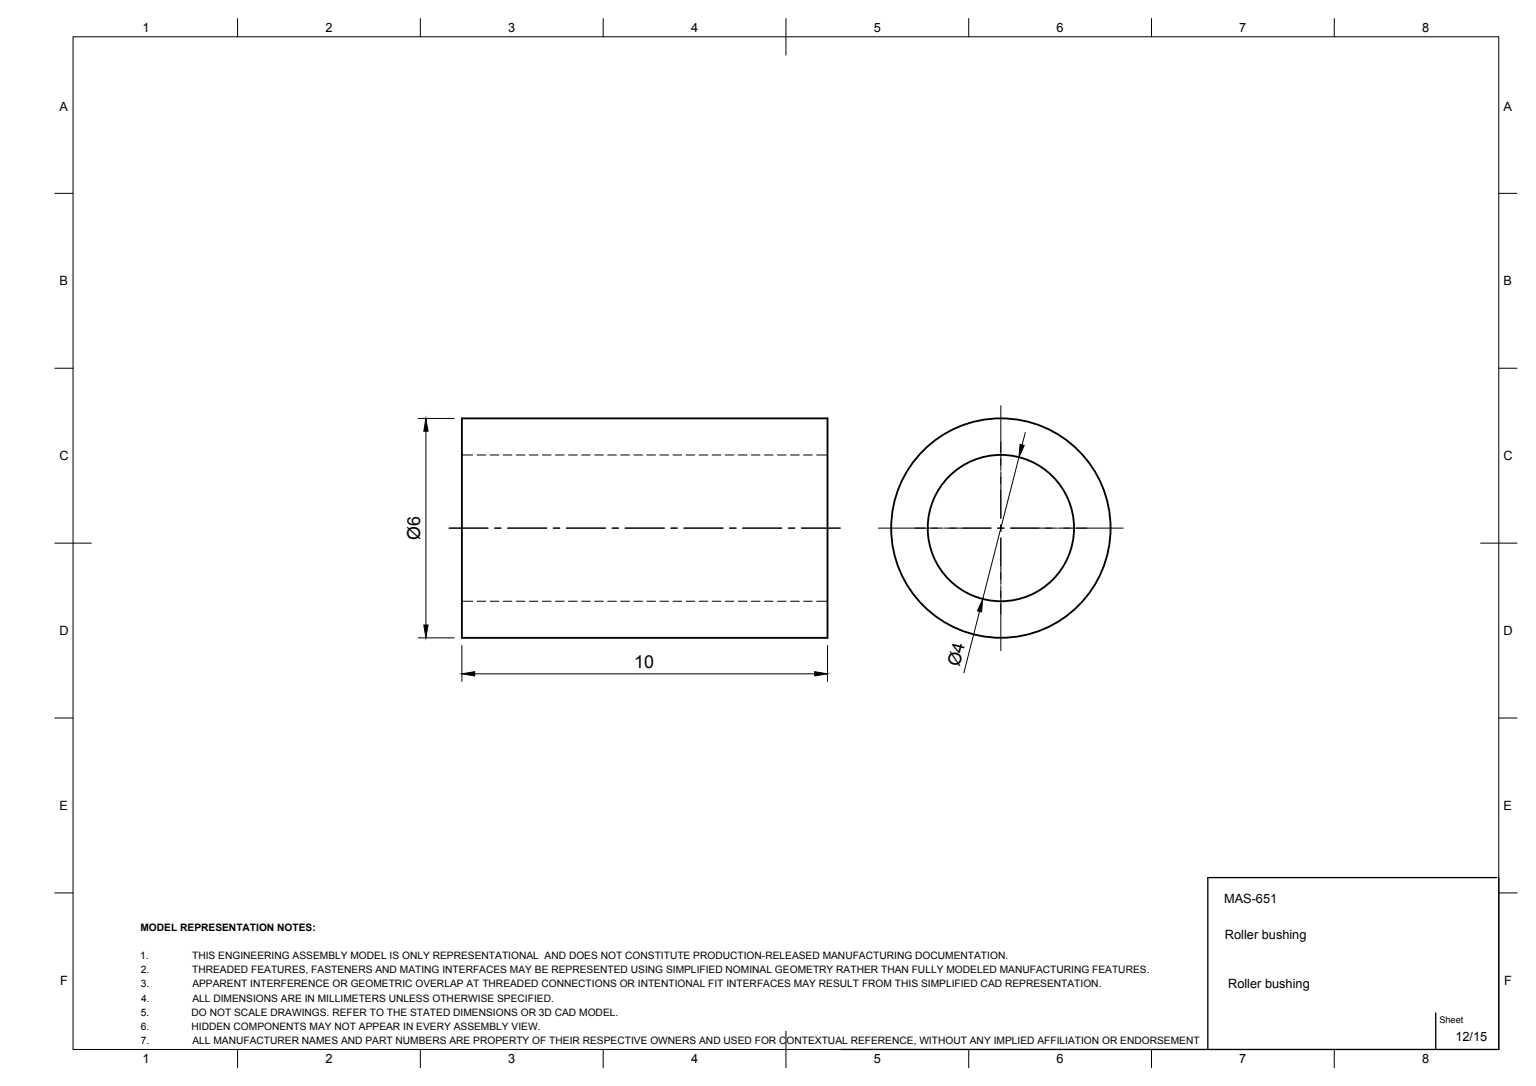
ISO-10303-21;
HEADER;
/* Generated by software containing ST-Developer
 * from STEP Tools, Inc. (www.steptools.com) 
 */

FILE_DESCRIPTION(
/* description */ ('Independent direct-acting normally-closed roller-plunger limit-switch
 CAD. Removable cover, insulated terminal supports, captured bus/conta
ct bridge, native Coil return spring, integral lower travel stop, reus
able instanced hardware and free roller. Manual geometric contact open
ing4mm; no snap-action/contact-force, electrical/current/voltage, envi
ronmental seal, safety-switch, wear, load or life certification. Exter
nal wiring and anchors omitted; fits and application engineering requi
red.'),
/* implementation_level */ '2;1');

FILE_NAME(
/* name */ 'Roller bushing.step',
/* time_stamp */ '2026-11-08T07:32:43-08:00',
/* author */ (''),
/* organization */ (''),
/* preprocessor_version */ 'ST-DEVELOPER v20.2',
/* originating_system */ 'Autodesk Translation Framework v15.17.0.0',
/* authorisation */ '');

FILE_SCHEMA (('AUTOMOTIVE_DESIGN { 1 0 10303 214 3 1 1 }'));
ENDSEC;

DATA;
#10=MECHANICAL_DESIGN_GEOMETRIC_PRESENTATION_REPRESENTATION('',(#185),#36482);
#151=SHAPE_REPRESENTATION_RELATIONSHIP('SRR','None',#36564,#168);
#168=ADVANCED_BREP_SHAPE_REPRESENTATION('',(#202),#36474);
#185=STYLED_ITEM('',(#36657),#202);
#202=MANIFOLD_SOLID_BREP('Body1',#9776);
#289=FACE_BOUND('',#1410,.T.);
#290=FACE_BOUND('',#1412,.T.);
#394=PLANE('',#10460);
#395=PLANE('',#10461);
#815=FACE_OUTER_BOUND('',#1407,.T.);
#816=FACE_OUTER_BOUND('',#1408,.T.);
#817=FACE_OUTER_BOUND('',#1409,.T.);
#818=FACE_OUTER_BOUND('',#1411,.T.);
#1407=EDGE_LOOP('',(#8038,#8039,#8040,#8041));
#1408=EDGE_LOOP('',(#8042,#8043,#8044,#8045));
#1409=EDGE_LOOP('',(#8046));
#1410=EDGE_LOOP('',(#8047));
#1411=EDGE_LOOP('',(#8048));
#1412=EDGE_LOOP('',(#8049));
#1695=CIRCLE('',#10455,0.2);
#1696=CIRCLE('',#10456,0.2);
#1697=CIRCLE('',#10458,0.3);
#1698=CIRCLE('',#10459,0.3);
#2855=LINE('',#29247,#3429);
#2856=LINE('',#29253,#3430);
#3429=VECTOR('',#12068,0.2);
#3430=VECTOR('',#12075,0.3);
#4275=VERTEX_POINT('',#29244);
#4276=VERTEX_POINT('',#29246);
#4277=VERTEX_POINT('',#29250);
#4278=VERTEX_POINT('',#29252);
#5575=EDGE_CURVE('',#4275,#4275,#1695,.T.);
#5576=EDGE_CURVE('',#4275,#4276,#2855,.T.);
#5577=EDGE_CURVE('',#4276,#4276,#1696,.T.);
#5578=EDGE_CURVE('',#4277,#4277,#1697,.T.);
#5579=EDGE_CURVE('',#4277,#4278,#2856,.T.);
#5580=EDGE_CURVE('',#4278,#4278,#1698,.T.);
#8038=ORIENTED_EDGE('',*,*,#5575,.F.);
#8039=ORIENTED_EDGE('',*,*,#5576,.T.);
#8040=ORIENTED_EDGE('',*,*,#5577,.T.);
#8041=ORIENTED_EDGE('',*,*,#5576,.F.);
#8042=ORIENTED_EDGE('',*,*,#5578,.F.);
#8043=ORIENTED_EDGE('',*,*,#5579,.T.);
#8044=ORIENTED_EDGE('',*,*,#5580,.T.);
#8045=ORIENTED_EDGE('',*,*,#5579,.F.);
#8046=ORIENTED_EDGE('',*,*,#5578,.T.);
#8047=ORIENTED_EDGE('',*,*,#5575,.T.);
#8048=ORIENTED_EDGE('',*,*,#5580,.F.);
#8049=ORIENTED_EDGE('',*,*,#5577,.F.);
#9122=CYLINDRICAL_SURFACE('',#10454,0.2);
#9123=CYLINDRICAL_SURFACE('',#10457,0.3);
#9605=ADVANCED_FACE('',(#815),#9122,.F.);
#9606=ADVANCED_FACE('',(#816),#9123,.T.);
#9607=ADVANCED_FACE('',(#817,#289),#394,.T.);
#9608=ADVANCED_FACE('',(#818,#290),#395,.F.);
#9776=CLOSED_SHELL('',(#9605,#9606,#9607,#9608));
#10453=AXIS2_PLACEMENT_3D('',#29242,#12062,#12063);
#10454=AXIS2_PLACEMENT_3D('',#29243,#12064,#12065);
#10455=AXIS2_PLACEMENT_3D('',#29245,#12066,#12067);
#10456=AXIS2_PLACEMENT_3D('',#29248,#12069,#12070);
#10457=AXIS2_PLACEMENT_3D('',#29249,#12071,#12072);
#10458=AXIS2_PLACEMENT_3D('',#29251,#12073,#12074);
#10459=AXIS2_PLACEMENT_3D('',#29254,#12076,#12077);
#10460=AXIS2_PLACEMENT_3D('',#29255,#12078,#12079);
#10461=AXIS2_PLACEMENT_3D('',#29256,#12080,#12081);
#12062=DIRECTION('axis',(0.,0.,1.));
#12063=DIRECTION('refdir',(1.,0.,0.));
#12064=DIRECTION('center_axis',(0.,0.,1.));
#12065=DIRECTION('ref_axis',(1.,0.,0.));
#12066=DIRECTION('center_axis',(0.,0.,-1.));
#12067=DIRECTION('ref_axis',(1.,0.,0.));
#12068=DIRECTION('',(0.,0.,-1.));
#12069=DIRECTION('center_axis',(0.,0.,-1.));
#12070=DIRECTION('ref_axis',(1.,0.,0.));
#12071=DIRECTION('center_axis',(0.,0.,1.));
#12072=DIRECTION('ref_axis',(1.,0.,0.));
#12073=DIRECTION('center_axis',(0.,0.,1.));
#12074=DIRECTION('ref_axis',(1.,0.,0.));
#12075=DIRECTION('',(0.,0.,-1.));
#12076=DIRECTION('center_axis',(0.,0.,1.));
#12077=DIRECTION('ref_axis',(1.,0.,0.));
#12078=DIRECTION('center_axis',(0.,0.,1.));
#12079=DIRECTION('ref_axis',(1.,0.,0.));
#12080=DIRECTION('center_axis',(0.,0.,1.));
#12081=DIRECTION('ref_axis',(1.,0.,0.));
#29242=CARTESIAN_POINT('',(0.,0.,0.));
#29243=CARTESIAN_POINT('Origin',(0.,0.,0.));
#29244=CARTESIAN_POINT('',(-0.2,-2.44929359829471E-17,1.));
#29245=CARTESIAN_POINT('Origin',(0.,0.,1.));
#29246=CARTESIAN_POINT('',(-0.2,-2.44929359829471E-17,0.));
#29247=CARTESIAN_POINT('',(-0.2,-2.44929359829471E-17,0.));
#29248=CARTESIAN_POINT('Origin',(0.,0.,0.));
#29249=CARTESIAN_POINT('Origin',(0.,0.,0.));
#29250=CARTESIAN_POINT('',(-0.3,-3.67394039744206E-17,1.));
#29251=CARTESIAN_POINT('Origin',(0.,0.,1.));
#29252=CARTESIAN_POINT('',(-0.3,-3.67394039744206E-17,0.));
#29253=CARTESIAN_POINT('',(-0.3,-3.67394039744206E-17,0.));
#29254=CARTESIAN_POINT('Origin',(0.,0.,0.));
#29255=CARTESIAN_POINT('Origin',(0.,0.,1.));
#29256=CARTESIAN_POINT('Origin',(0.,0.,0.));
#36455=UNCERTAINTY_MEASURE_WITH_UNIT(LENGTH_MEASURE(0.001),#36483,
'DISTANCE_ACCURACY_VALUE',
'Maximum model space distance between geometric entities at asserted c
onnectivities');
#36463=UNCERTAINTY_MEASURE_WITH_UNIT(LENGTH_MEASURE(0.001),#36483,
'DISTANCE_ACCURACY_VALUE',
'Maximum model space distance between geometric entities at asserted c
onnectivities');
#36474=(
GEOMETRIC_REPRESENTATION_CONTEXT(3)
GLOBAL_UNCERTAINTY_ASSIGNED_CONTEXT((#36455))
GLOBAL_UNIT_ASSIGNED_CONTEXT((#36483,#36485,#36486))
REPRESENTATION_CONTEXT('','3D')
);
#36482=(
GEOMETRIC_REPRESENTATION_CONTEXT(3)
GLOBAL_UNCERTAINTY_ASSIGNED_CONTEXT((#36463))
GLOBAL_UNIT_ASSIGNED_CONTEXT((#36483,#36485,#36486))
REPRESENTATION_CONTEXT('','3D')
);
#36483=(
LENGTH_UNIT()
NAMED_UNIT(*)
SI_UNIT(.CENTI.,.METRE.)
);
#36485=(
NAMED_UNIT(*)
PLANE_ANGLE_UNIT()
SI_UNIT($,.RADIAN.)
);
#36486=(
NAMED_UNIT(*)
SI_UNIT($,.STERADIAN.)
SOLID_ANGLE_UNIT()
);
#36497=SHAPE_DEFINITION_REPRESENTATION(#36515,#36564);
#36515=PRODUCT_DEFINITION_SHAPE('',$,#36583);
#36564=SHAPE_REPRESENTATION('',(#10453),#36474);
#36572=PRODUCT_DEFINITION_CONTEXT('part definition',#36628,'design');
#36583=PRODUCT_DEFINITION('Roller bushing','Roller bushing',#36601,#36572);
#36601=PRODUCT_DEFINITION_FORMATION('',$,#36640);
#36628=APPLICATION_CONTEXT(
'Core Data for Automotive Mechanical Design Process');
#36629=PRODUCT_CONTEXT('part definition',#36628,'mechanical');
#36640=PRODUCT('Roller bushing','Roller bushing',$,(#36629));
#36657=PRESENTATION_STYLE_ASSIGNMENT((#36671));
#36671=SURFACE_STYLE_USAGE(.BOTH.,#36685);
#36685=SURFACE_SIDE_STYLE('',(#36699));
#36699=SURFACE_STYLE_FILL_AREA(#36713);
#36713=FILL_AREA_STYLE('Bearing gray',(#36727));
#36727=FILL_AREA_STYLE_COLOUR('Bearing gray',#36741);
#36741=COLOUR_RGB('Bearing gray',0.725490196078431,0.752941176470588,0.792156862745098);
ENDSEC;
END-ISO-10303-21;
